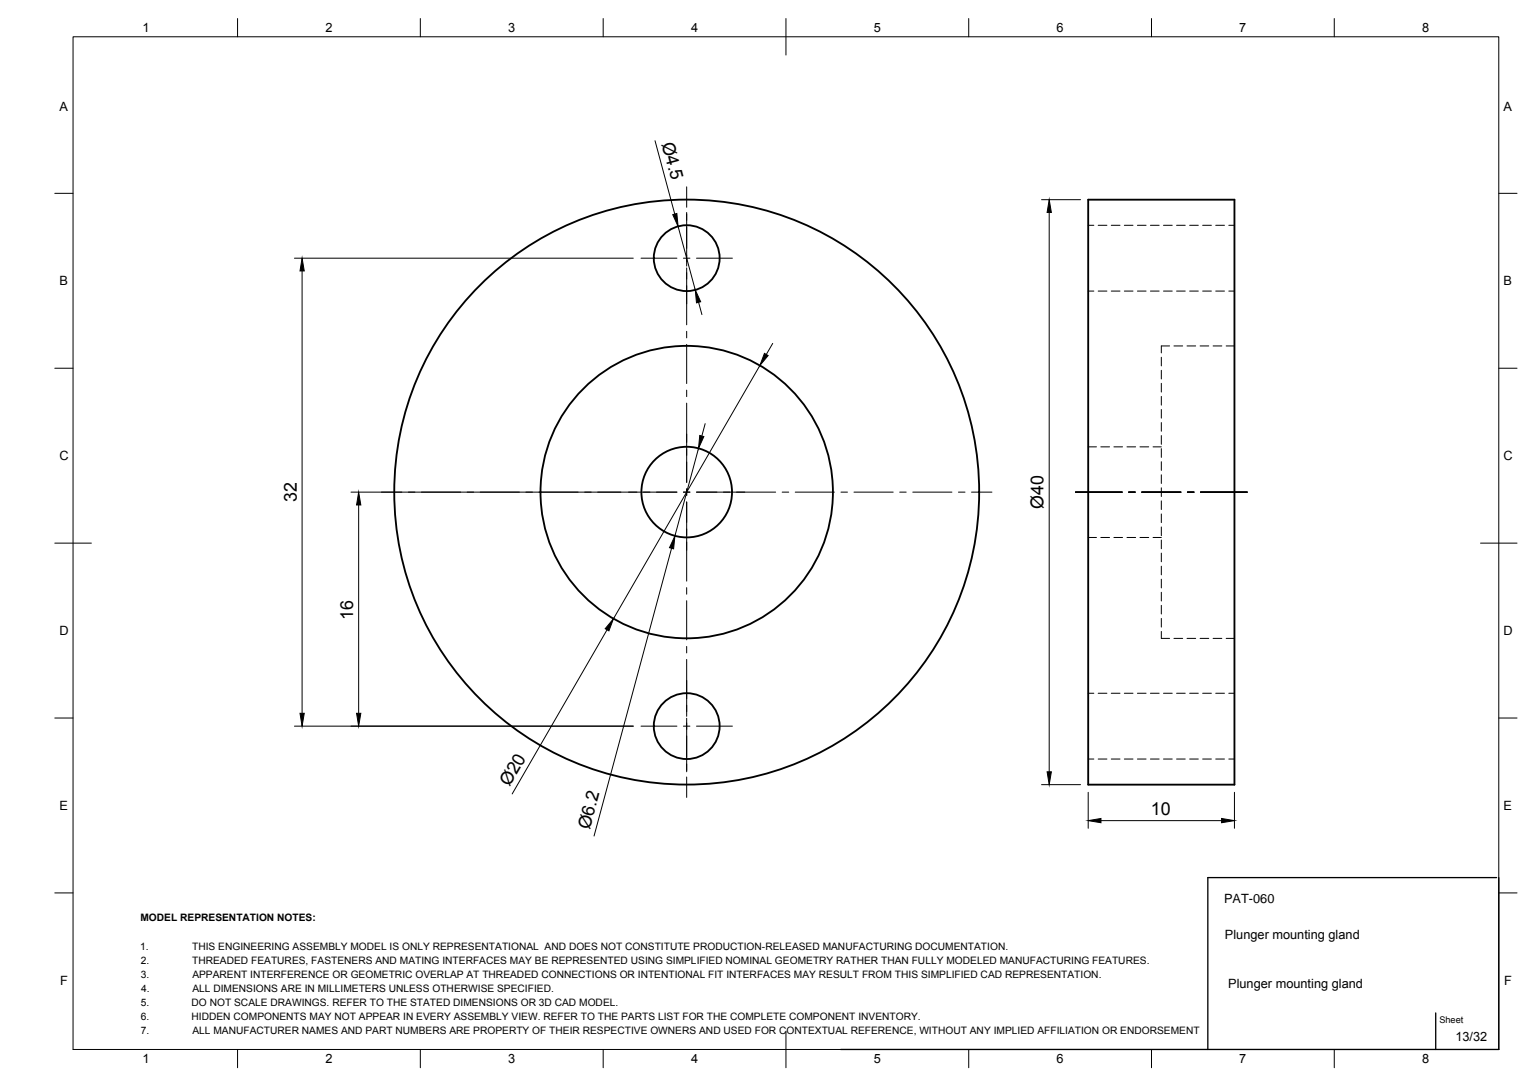
ISO-10303-21;
HEADER;
/* Generated by software containing ST-Developer
 * from STEP Tools, Inc. (www.steptools.com) 
 */

FILE_DESCRIPTION(
/* description */ ('Indexing fixture plate with plunger'),
/* implementation_level */ '2;1');

FILE_NAME(
/* name */ 'Plunger mounting gland.step',
/* time_stamp */ '2026-10-28T03:23:41-07:00',
/* author */ (''),
/* organization */ (''),
/* preprocessor_version */ 'ST-DEVELOPER v20.2',
/* originating_system */ 'Autodesk Translation Framework v15.17.0.0',
/* authorisation */ '');

FILE_SCHEMA (('AUTOMOTIVE_DESIGN { 1 0 10303 214 3 1 1 }'));
ENDSEC;

DATA;
#10=MECHANICAL_DESIGN_GEOMETRIC_PRESENTATION_REPRESENTATION('',(#325),#10020);
#271=SHAPE_REPRESENTATION_RELATIONSHIP('SRR','None',#10145,#298);
#298=ADVANCED_BREP_SHAPE_REPRESENTATION('',(#361),#9998);
#325=STYLED_ITEM('',(#10354),#361);
#361=MANIFOLD_SOLID_BREP('Body1',#4579);
#418=FACE_BOUND('',#1040,.T.);
#419=FACE_BOUND('',#1044,.T.);
#420=FACE_BOUND('',#1045,.T.);
#421=FACE_BOUND('',#1046,.T.);
#422=FACE_BOUND('',#1048,.T.);
#423=FACE_BOUND('',#1049,.T.);
#424=FACE_BOUND('',#1050,.T.);
#562=PLANE('',#5024);
#563=PLANE('',#5031);
#564=PLANE('',#5032);
#719=FACE_OUTER_BOUND('',#1036,.T.);
#720=FACE_OUTER_BOUND('',#1037,.T.);
#721=FACE_OUTER_BOUND('',#1038,.T.);
#722=FACE_OUTER_BOUND('',#1039,.T.);
#723=FACE_OUTER_BOUND('',#1041,.T.);
#724=FACE_OUTER_BOUND('',#1042,.T.);
#725=FACE_OUTER_BOUND('',#1043,.T.);
#726=FACE_OUTER_BOUND('',#1047,.T.);
#1036=EDGE_LOOP('',(#3245,#3246,#3247,#3248));
#1037=EDGE_LOOP('',(#3249,#3250,#3251,#3252));
#1038=EDGE_LOOP('',(#3253,#3254,#3255,#3256));
#1039=EDGE_LOOP('',(#3257));
#1040=EDGE_LOOP('',(#3258));
#1041=EDGE_LOOP('',(#3259,#3260,#3261,#3262));
#1042=EDGE_LOOP('',(#3263,#3264,#3265,#3266));
#1043=EDGE_LOOP('',(#3267));
#1044=EDGE_LOOP('',(#3268));
#1045=EDGE_LOOP('',(#3269));
#1046=EDGE_LOOP('',(#3270));
#1047=EDGE_LOOP('',(#3271));
#1048=EDGE_LOOP('',(#3272));
#1049=EDGE_LOOP('',(#3273));
#1050=EDGE_LOOP('',(#3274));
#1430=LINE('',#7402,#1650);
#1431=LINE('',#7408,#1651);
#1432=LINE('',#7414,#1652);
#1433=LINE('',#7421,#1653);
#1434=LINE('',#7427,#1654);
#1650=VECTOR('',#5831,0.225);
#1651=VECTOR('',#5838,0.225);
#1652=VECTOR('',#5845,0.999999999999999);
#1653=VECTOR('',#5854,0.31);
#1654=VECTOR('',#5861,2.);
#1880=CIRCLE('',#5016,0.225);
#1881=CIRCLE('',#5017,0.225);
#1882=CIRCLE('',#5019,0.225);
#1883=CIRCLE('',#5020,0.225);
#1884=CIRCLE('',#5022,0.999999999999999);
#1885=CIRCLE('',#5023,0.999999999999999);
#1886=CIRCLE('',#5025,0.31);
#1887=CIRCLE('',#5027,0.31);
#1888=CIRCLE('',#5029,2.);
#1889=CIRCLE('',#5030,2.);
#2196=VERTEX_POINT('',#7399);
#2197=VERTEX_POINT('',#7401);
#2198=VERTEX_POINT('',#7405);
#2199=VERTEX_POINT('',#7407);
#2200=VERTEX_POINT('',#7411);
#2201=VERTEX_POINT('',#7413);
#2202=VERTEX_POINT('',#7417);
#2203=VERTEX_POINT('',#7420);
#2204=VERTEX_POINT('',#7424);
#2205=VERTEX_POINT('',#7426);
#2602=EDGE_CURVE('',#2196,#2196,#1880,.T.);
#2603=EDGE_CURVE('',#2196,#2197,#1430,.T.);
#2604=EDGE_CURVE('',#2197,#2197,#1881,.T.);
#2605=EDGE_CURVE('',#2198,#2198,#1882,.T.);
#2606=EDGE_CURVE('',#2198,#2199,#1431,.T.);
#2607=EDGE_CURVE('',#2199,#2199,#1883,.T.);
#2608=EDGE_CURVE('',#2200,#2200,#1884,.T.);
#2609=EDGE_CURVE('',#2200,#2201,#1432,.T.);
#2610=EDGE_CURVE('',#2201,#2201,#1885,.T.);
#2611=EDGE_CURVE('',#2202,#2202,#1886,.T.);
#2612=EDGE_CURVE('',#2202,#2203,#1433,.T.);
#2613=EDGE_CURVE('',#2203,#2203,#1887,.T.);
#2614=EDGE_CURVE('',#2204,#2204,#1888,.T.);
#2615=EDGE_CURVE('',#2204,#2205,#1434,.T.);
#2616=EDGE_CURVE('',#2205,#2205,#1889,.T.);
#3245=ORIENTED_EDGE('',*,*,#2602,.F.);
#3246=ORIENTED_EDGE('',*,*,#2603,.T.);
#3247=ORIENTED_EDGE('',*,*,#2604,.F.);
#3248=ORIENTED_EDGE('',*,*,#2603,.F.);
#3249=ORIENTED_EDGE('',*,*,#2605,.F.);
#3250=ORIENTED_EDGE('',*,*,#2606,.T.);
#3251=ORIENTED_EDGE('',*,*,#2607,.F.);
#3252=ORIENTED_EDGE('',*,*,#2606,.F.);
#3253=ORIENTED_EDGE('',*,*,#2608,.F.);
#3254=ORIENTED_EDGE('',*,*,#2609,.T.);
#3255=ORIENTED_EDGE('',*,*,#2610,.F.);
#3256=ORIENTED_EDGE('',*,*,#2609,.F.);
#3257=ORIENTED_EDGE('',*,*,#2608,.T.);
#3258=ORIENTED_EDGE('',*,*,#2611,.F.);
#3259=ORIENTED_EDGE('',*,*,#2611,.T.);
#3260=ORIENTED_EDGE('',*,*,#2612,.T.);
#3261=ORIENTED_EDGE('',*,*,#2613,.T.);
#3262=ORIENTED_EDGE('',*,*,#2612,.F.);
#3263=ORIENTED_EDGE('',*,*,#2614,.F.);
#3264=ORIENTED_EDGE('',*,*,#2615,.T.);
#3265=ORIENTED_EDGE('',*,*,#2616,.T.);
#3266=ORIENTED_EDGE('',*,*,#2615,.F.);
#3267=ORIENTED_EDGE('',*,*,#2614,.T.);
#3268=ORIENTED_EDGE('',*,*,#2604,.T.);
#3269=ORIENTED_EDGE('',*,*,#2607,.T.);
#3270=ORIENTED_EDGE('',*,*,#2610,.T.);
#3271=ORIENTED_EDGE('',*,*,#2616,.F.);
#3272=ORIENTED_EDGE('',*,*,#2602,.T.);
#3273=ORIENTED_EDGE('',*,*,#2605,.T.);
#3274=ORIENTED_EDGE('',*,*,#2613,.F.);
#4191=CYLINDRICAL_SURFACE('',#5015,0.225);
#4192=CYLINDRICAL_SURFACE('',#5018,0.225);
#4193=CYLINDRICAL_SURFACE('',#5021,0.999999999999999);
#4194=CYLINDRICAL_SURFACE('',#5026,0.31);
#4195=CYLINDRICAL_SURFACE('',#5028,2.);
#4334=ADVANCED_FACE('',(#719),#4191,.F.);
#4335=ADVANCED_FACE('',(#720),#4192,.F.);
#4336=ADVANCED_FACE('',(#721),#4193,.F.);
#4337=ADVANCED_FACE('',(#722,#418),#562,.T.);
#4338=ADVANCED_FACE('',(#723),#4194,.F.);
#4339=ADVANCED_FACE('',(#724),#4195,.T.);
#4340=ADVANCED_FACE('',(#725,#419,#420,#421),#563,.T.);
#4341=ADVANCED_FACE('',(#726,#422,#423,#424),#564,.F.);
#4579=CLOSED_SHELL('',(#4334,#4335,#4336,#4337,#4338,#4339,#4340,#4341));
#5014=AXIS2_PLACEMENT_3D('',#7397,#5825,#5826);
#5015=AXIS2_PLACEMENT_3D('',#7398,#5827,#5828);
#5016=AXIS2_PLACEMENT_3D('',#7400,#5829,#5830);
#5017=AXIS2_PLACEMENT_3D('',#7403,#5832,#5833);
#5018=AXIS2_PLACEMENT_3D('',#7404,#5834,#5835);
#5019=AXIS2_PLACEMENT_3D('',#7406,#5836,#5837);
#5020=AXIS2_PLACEMENT_3D('',#7409,#5839,#5840);
#5021=AXIS2_PLACEMENT_3D('',#7410,#5841,#5842);
#5022=AXIS2_PLACEMENT_3D('',#7412,#5843,#5844);
#5023=AXIS2_PLACEMENT_3D('',#7415,#5846,#5847);
#5024=AXIS2_PLACEMENT_3D('',#7416,#5848,#5849);
#5025=AXIS2_PLACEMENT_3D('',#7418,#5850,#5851);
#5026=AXIS2_PLACEMENT_3D('',#7419,#5852,#5853);
#5027=AXIS2_PLACEMENT_3D('',#7422,#5855,#5856);
#5028=AXIS2_PLACEMENT_3D('',#7423,#5857,#5858);
#5029=AXIS2_PLACEMENT_3D('',#7425,#5859,#5860);
#5030=AXIS2_PLACEMENT_3D('',#7428,#5862,#5863);
#5031=AXIS2_PLACEMENT_3D('',#7429,#5864,#5865);
#5032=AXIS2_PLACEMENT_3D('',#7430,#5866,#5867);
#5825=DIRECTION('axis',(0.,0.,1.));
#5826=DIRECTION('refdir',(1.,0.,0.));
#5827=DIRECTION('center_axis',(0.,0.,1.));
#5828=DIRECTION('ref_axis',(1.,0.,0.));
#5829=DIRECTION('center_axis',(0.,0.,1.));
#5830=DIRECTION('ref_axis',(1.,0.,0.));
#5831=DIRECTION('',(0.,0.,1.));
#5832=DIRECTION('center_axis',(0.,0.,-1.));
#5833=DIRECTION('ref_axis',(1.,0.,0.));
#5834=DIRECTION('center_axis',(0.,0.,1.));
#5835=DIRECTION('ref_axis',(1.,0.,0.));
#5836=DIRECTION('center_axis',(0.,0.,1.));
#5837=DIRECTION('ref_axis',(1.,0.,0.));
#5838=DIRECTION('',(0.,0.,1.));
#5839=DIRECTION('center_axis',(0.,0.,-1.));
#5840=DIRECTION('ref_axis',(1.,0.,0.));
#5841=DIRECTION('center_axis',(0.,0.,1.));
#5842=DIRECTION('ref_axis',(1.,0.,0.));
#5843=DIRECTION('center_axis',(0.,0.,1.));
#5844=DIRECTION('ref_axis',(1.,0.,0.));
#5845=DIRECTION('',(0.,0.,1.));
#5846=DIRECTION('center_axis',(0.,0.,-1.));
#5847=DIRECTION('ref_axis',(1.,0.,0.));
#5848=DIRECTION('center_axis',(0.,0.,1.));
#5849=DIRECTION('ref_axis',(1.,0.,0.));
#5850=DIRECTION('center_axis',(0.,0.,1.));
#5851=DIRECTION('ref_axis',(1.,0.,0.));
#5852=DIRECTION('center_axis',(0.,0.,1.));
#5853=DIRECTION('ref_axis',(1.,0.,0.));
#5854=DIRECTION('',(0.,0.,-1.));
#5855=DIRECTION('center_axis',(0.,0.,-1.));
#5856=DIRECTION('ref_axis',(1.,0.,0.));
#5857=DIRECTION('center_axis',(0.,0.,1.));
#5858=DIRECTION('ref_axis',(1.,0.,0.));
#5859=DIRECTION('center_axis',(0.,0.,1.));
#5860=DIRECTION('ref_axis',(1.,0.,0.));
#5861=DIRECTION('',(0.,0.,-1.));
#5862=DIRECTION('center_axis',(0.,0.,1.));
#5863=DIRECTION('ref_axis',(1.,0.,0.));
#5864=DIRECTION('center_axis',(0.,0.,1.));
#5865=DIRECTION('ref_axis',(1.,0.,0.));
#5866=DIRECTION('center_axis',(0.,0.,1.));
#5867=DIRECTION('ref_axis',(1.,0.,0.));
#7397=CARTESIAN_POINT('',(0.,0.,0.));
#7398=CARTESIAN_POINT('Origin',(7.2,1.6,-0.1));
#7399=CARTESIAN_POINT('',(6.975,1.6,0.));
#7400=CARTESIAN_POINT('Origin',(7.2,1.6,0.));
#7401=CARTESIAN_POINT('',(6.975,1.6,1.));
#7402=CARTESIAN_POINT('',(6.975,1.6,-0.1));
#7403=CARTESIAN_POINT('Origin',(7.2,1.6,1.));
#7404=CARTESIAN_POINT('Origin',(7.2,-1.6,-0.1));
#7405=CARTESIAN_POINT('',(6.975,-1.6,0.));
#7406=CARTESIAN_POINT('Origin',(7.2,-1.6,0.));
#7407=CARTESIAN_POINT('',(6.975,-1.6,1.));
#7408=CARTESIAN_POINT('',(6.975,-1.6,-0.1));
#7409=CARTESIAN_POINT('Origin',(7.2,-1.6,1.));
#7410=CARTESIAN_POINT('Origin',(7.2,0.,0.5));
#7411=CARTESIAN_POINT('',(6.2,-1.22464679914735E-16,0.5));
#7412=CARTESIAN_POINT('Origin',(7.2,0.,0.5));
#7413=CARTESIAN_POINT('',(6.2,1.22464679914735E-16,1.));
#7414=CARTESIAN_POINT('',(6.2,-1.22464679914735E-16,0.5));
#7415=CARTESIAN_POINT('Origin',(7.2,0.,1.));
#7416=CARTESIAN_POINT('Origin',(7.2,0.,0.5));
#7417=CARTESIAN_POINT('',(6.89,-3.79640507735679E-17,0.5));
#7418=CARTESIAN_POINT('Origin',(7.2,0.,0.5));
#7419=CARTESIAN_POINT('Origin',(7.2,0.,0.));
#7420=CARTESIAN_POINT('',(6.89,-3.79640507735679E-17,0.));
#7421=CARTESIAN_POINT('',(6.89,-3.79640507735679E-17,0.));
#7422=CARTESIAN_POINT('Origin',(7.2,0.,0.));
#7423=CARTESIAN_POINT('Origin',(7.2,0.,0.));
#7424=CARTESIAN_POINT('',(5.2,-2.44929359829471E-16,1.));
#7425=CARTESIAN_POINT('Origin',(7.2,0.,1.));
#7426=CARTESIAN_POINT('',(5.2,-2.44929359829471E-16,0.));
#7427=CARTESIAN_POINT('',(5.2,-2.44929359829471E-16,0.));
#7428=CARTESIAN_POINT('Origin',(7.2,0.,0.));
#7429=CARTESIAN_POINT('Origin',(7.2,0.,1.));
#7430=CARTESIAN_POINT('Origin',(7.2,0.,0.));
#9965=UNCERTAINTY_MEASURE_WITH_UNIT(LENGTH_MEASURE(0.001),#10021,
'DISTANCE_ACCURACY_VALUE',
'Maximum model space distance between geometric entities at asserted c
onnectivities');
#9987=UNCERTAINTY_MEASURE_WITH_UNIT(LENGTH_MEASURE(0.001),#10021,
'DISTANCE_ACCURACY_VALUE',
'Maximum model space distance between geometric entities at asserted c
onnectivities');
#9998=(
GEOMETRIC_REPRESENTATION_CONTEXT(3)
GLOBAL_UNCERTAINTY_ASSIGNED_CONTEXT((#9965))
GLOBAL_UNIT_ASSIGNED_CONTEXT((#10021,#10023,#10024))
REPRESENTATION_CONTEXT('','3D')
);
#10020=(
GEOMETRIC_REPRESENTATION_CONTEXT(3)
GLOBAL_UNCERTAINTY_ASSIGNED_CONTEXT((#9987))
GLOBAL_UNIT_ASSIGNED_CONTEXT((#10021,#10023,#10024))
REPRESENTATION_CONTEXT('','3D')
);
#10021=(
LENGTH_UNIT()
NAMED_UNIT(*)
SI_UNIT(.CENTI.,.METRE.)
);
#10023=(
NAMED_UNIT(*)
PLANE_ANGLE_UNIT()
SI_UNIT($,.RADIAN.)
);
#10024=(
NAMED_UNIT(*)
SI_UNIT($,.STERADIAN.)
SOLID_ANGLE_UNIT()
);
#10035=SHAPE_DEFINITION_REPRESENTATION(#10067,#10145);
#10067=PRODUCT_DEFINITION_SHAPE('',$,#10178);
#10145=SHAPE_REPRESENTATION('',(#5014),#9998);
#10167=PRODUCT_DEFINITION_CONTEXT('part definition',#10265,'design');
#10178=PRODUCT_DEFINITION('Plunger mounting gland',
'Plunger mounting gland',#10210,#10167);
#10210=PRODUCT_DEFINITION_FORMATION('',$,#10277);
#10265=APPLICATION_CONTEXT(
'Core Data for Automotive Mechanical Design Process');
#10266=PRODUCT_CONTEXT('part definition',#10265,'mechanical');
#10277=PRODUCT('Plunger mounting gland','Plunger mounting gland',
'Plunger mounting gland',(#10266));
#10348=COLOUR_RGB('Light Blue',0.38,0.62,0.78);
#10349=FILL_AREA_STYLE_COLOUR('',#10348);
#10350=FILL_AREA_STYLE('',(#10349));
#10351=SURFACE_STYLE_FILL_AREA(#10350);
#10352=SURFACE_SIDE_STYLE('',(#10351));
#10353=SURFACE_STYLE_USAGE(.BOTH.,#10352);
#10354=PRESENTATION_STYLE_ASSIGNMENT((#10353));
ENDSEC;
END-ISO-10303-21;
